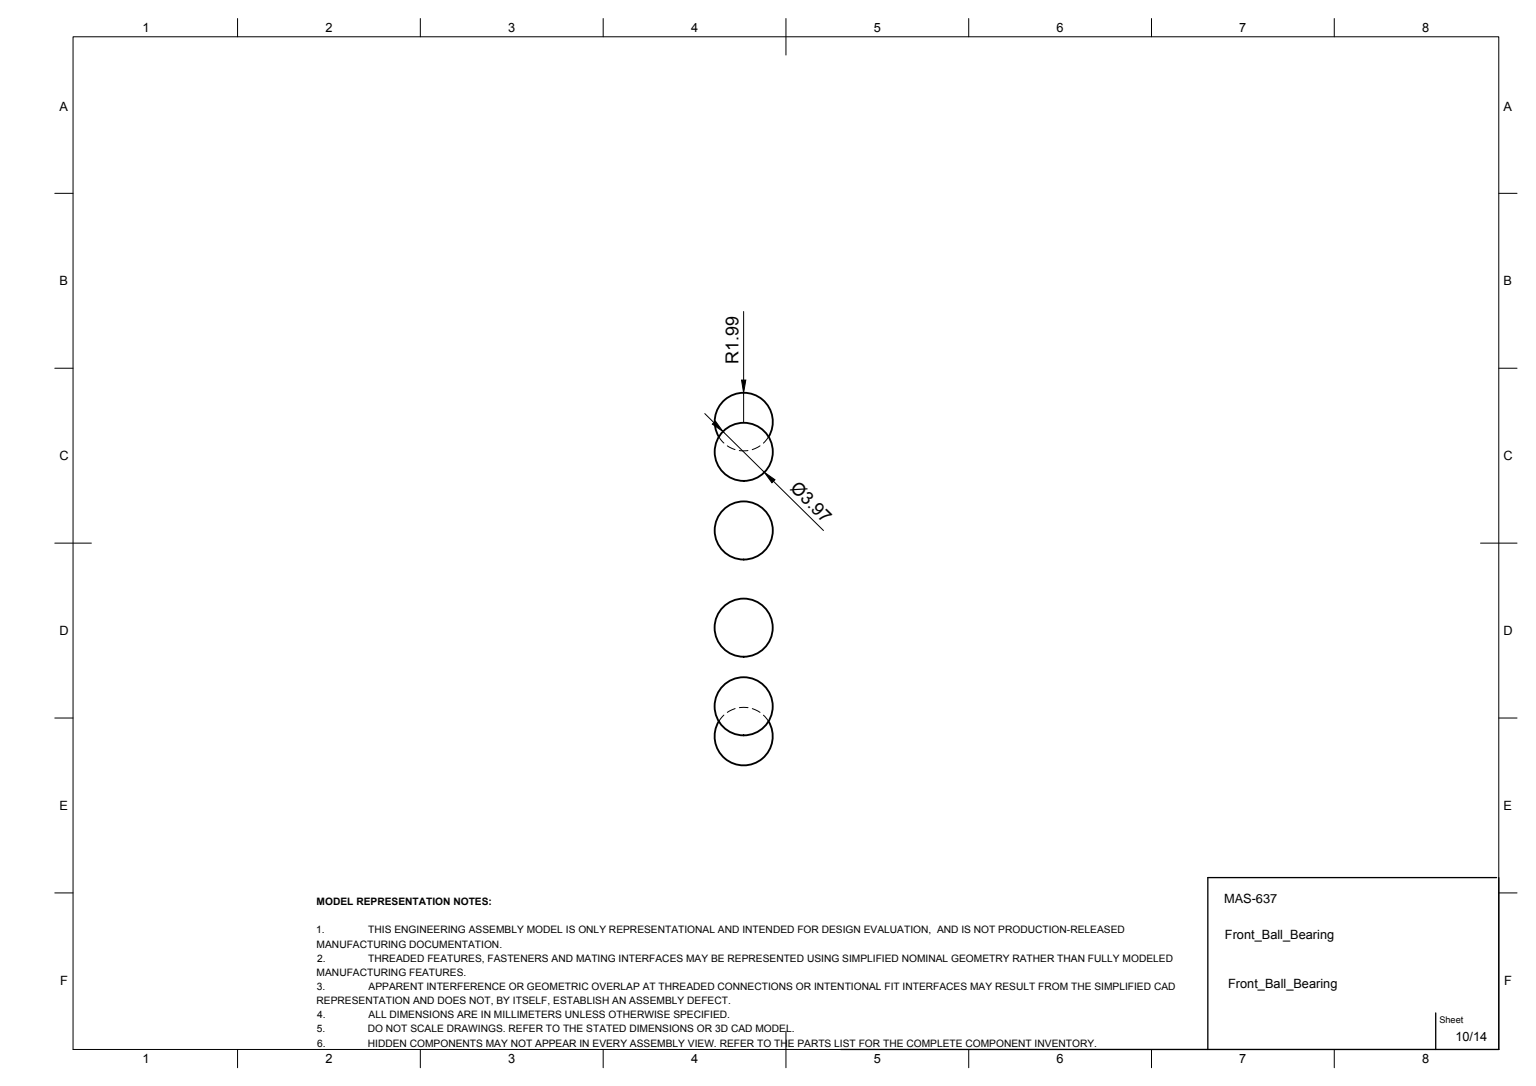
ISO-10303-21;
HEADER;
FILE_DESCRIPTION((''),'2;1');
FILE_NAME('Front_Ball_Bearing.step','2026-10-09T10:11:57-07:00',(''),(''),'','','');
FILE_SCHEMA (('AUTOMOTIVE_DESIGN { 1 0 10303 214 3 1 1 }'));
ENDSEC;
DATA;
#10=MECHANICAL_DESIGN_GEOMETRIC_PRESENTATION_REPRESENTATION('',(#133,#134,#135,#136,#137,#138,#139,#140,#141,#142),#13510);
#74=SPHERICAL_SURFACE('',#8349,1.985) ;
#75=SPHERICAL_SURFACE('',#8351,1.985) ;
#76=SPHERICAL_SURFACE('',#8353,1.985) ;
#77=SPHERICAL_SURFACE('',#8355,1.985) ;
#78=SPHERICAL_SURFACE('',#8357,1.985) ;
#79=SPHERICAL_SURFACE('',#8359,1.985) ;
#80=SPHERICAL_SURFACE('',#8361,1.985) ;
#81=SPHERICAL_SURFACE('',#8363,1.985) ;
#82=SPHERICAL_SURFACE('',#8365,1.985) ;
#83=SPHERICAL_SURFACE('',#8367,1.985) ;
#103=SHAPE_REPRESENTATION_RELATIONSHIP('SRR','None',#13573,#118) ;
#118=ADVANCED_BREP_SHAPE_REPRESENTATION('',(#165,#166,#167,#168,#169,#170,
#171,#172,#173,#174),#13505) ;
#133=STYLED_ITEM('',(#13650),#165) ;
#134=STYLED_ITEM('',(#13650),#166) ;
#135=STYLED_ITEM('',(#13650),#167) ;
#136=STYLED_ITEM('',(#13650),#168) ;
#137=STYLED_ITEM('',(#13650),#169) ;
#138=STYLED_ITEM('',(#13650),#170) ;
#139=STYLED_ITEM('',(#13650),#171) ;
#140=STYLED_ITEM('',(#13650),#172) ;
#141=STYLED_ITEM('',(#13650),#173) ;
#142=STYLED_ITEM('',(#13650),#174) ;
#165=MANIFOLD_SOLID_BREP('Body1',#7382) ;
#166=MANIFOLD_SOLID_BREP('Body2',#7383) ;
#167=MANIFOLD_SOLID_BREP('Body3',#7384) ;
#168=MANIFOLD_SOLID_BREP('Body4',#7385) ;
#169=MANIFOLD_SOLID_BREP('Body5',#7386) ;
#170=MANIFOLD_SOLID_BREP('Body6',#7387) ;
#171=MANIFOLD_SOLID_BREP('Body7',#7388) ;
#172=MANIFOLD_SOLID_BREP('Body8',#7389) ;
#173=MANIFOLD_SOLID_BREP('Body9',#7390) ;
#174=MANIFOLD_SOLID_BREP('Body10',#7391) ;
#1035=FACE_OUTER_BOUND('',#1550,.T.) ;
#1036=FACE_OUTER_BOUND('',#1551,.T.) ;
#1037=FACE_OUTER_BOUND('',#1552,.T.) ;
#1038=FACE_OUTER_BOUND('',#1553,.T.) ;
#1039=FACE_OUTER_BOUND('',#1554,.T.) ;
#1040=FACE_OUTER_BOUND('',#1555,.T.) ;
#1041=FACE_OUTER_BOUND('',#1556,.T.) ;
#1042=FACE_OUTER_BOUND('',#1557,.T.) ;
#1043=FACE_OUTER_BOUND('',#1558,.T.) ;
#1044=FACE_OUTER_BOUND('',#1559,.T.) ;
#1550=EDGE_LOOP('',(#6584,#6585)) ;
#1551=EDGE_LOOP('',(#6586,#6587)) ;
#1552=EDGE_LOOP('',(#6588,#6589)) ;
#1553=EDGE_LOOP('',(#6590,#6591)) ;
#1554=EDGE_LOOP('',(#6592,#6593)) ;
#1555=EDGE_LOOP('',(#6594,#6595)) ;
#1556=EDGE_LOOP('',(#6596,#6597)) ;
#1557=EDGE_LOOP('',(#6598,#6599)) ;
#1558=EDGE_LOOP('',(#6600,#6601)) ;
#1559=EDGE_LOOP('',(#6602,#6603)) ;
#3031=CIRCLE('',#8350,1.985) ;
#3032=CIRCLE('',#8352,1.985) ;
#3033=CIRCLE('',#8354,1.985) ;
#3034=CIRCLE('',#8356,1.985) ;
#3035=CIRCLE('',#8358,1.985) ;
#3036=CIRCLE('',#8360,1.985) ;
#3037=CIRCLE('',#8362,1.985) ;
#3038=CIRCLE('',#8364,1.985) ;
#3039=CIRCLE('',#8366,1.985) ;
#3040=CIRCLE('',#8368,1.985) ;
#3692=VERTEX_POINT('',#13123) ;
#3693=VERTEX_POINT('',#13124) ;
#3694=VERTEX_POINT('',#13127) ;
#3695=VERTEX_POINT('',#13128) ;
#3696=VERTEX_POINT('',#13131) ;
#3697=VERTEX_POINT('',#13132) ;
#3698=VERTEX_POINT('',#13135) ;
#3699=VERTEX_POINT('',#13136) ;
#3700=VERTEX_POINT('',#13139) ;
#3701=VERTEX_POINT('',#13140) ;
#3702=VERTEX_POINT('',#13143) ;
#3703=VERTEX_POINT('',#13144) ;
#3704=VERTEX_POINT('',#13147) ;
#3705=VERTEX_POINT('',#13148) ;
#3706=VERTEX_POINT('',#13151) ;
#3707=VERTEX_POINT('',#13152) ;
#3708=VERTEX_POINT('',#13155) ;
#3709=VERTEX_POINT('',#13156) ;
#3710=VERTEX_POINT('',#13159) ;
#3711=VERTEX_POINT('',#13160) ;
#4679=EDGE_CURVE('',#3692,#3693,#3031,.T.) ;
#4680=EDGE_CURVE('',#3694,#3695,#3032,.T.) ;
#4681=EDGE_CURVE('',#3696,#3697,#3033,.T.) ;
#4682=EDGE_CURVE('',#3698,#3699,#3034,.T.) ;
#4683=EDGE_CURVE('',#3700,#3701,#3035,.T.) ;
#4684=EDGE_CURVE('',#3702,#3703,#3036,.T.) ;
#4685=EDGE_CURVE('',#3704,#3705,#3037,.T.) ;
#4686=EDGE_CURVE('',#3706,#3707,#3038,.T.) ;
#4687=EDGE_CURVE('',#3708,#3709,#3039,.T.) ;
#4688=EDGE_CURVE('',#3710,#3711,#3040,.T.) ;
#6584=ORIENTED_EDGE('',*,*,#4679,.T.) ;
#6585=ORIENTED_EDGE('',*,*,#4679,.F.) ;
#6586=ORIENTED_EDGE('',*,*,#4680,.T.) ;
#6587=ORIENTED_EDGE('',*,*,#4680,.F.) ;
#6588=ORIENTED_EDGE('',*,*,#4681,.T.) ;
#6589=ORIENTED_EDGE('',*,*,#4681,.F.) ;
#6590=ORIENTED_EDGE('',*,*,#4682,.T.) ;
#6591=ORIENTED_EDGE('',*,*,#4682,.F.) ;
#6592=ORIENTED_EDGE('',*,*,#4683,.T.) ;
#6593=ORIENTED_EDGE('',*,*,#4683,.F.) ;
#6594=ORIENTED_EDGE('',*,*,#4684,.T.) ;
#6595=ORIENTED_EDGE('',*,*,#4684,.F.) ;
#6596=ORIENTED_EDGE('',*,*,#4685,.T.) ;
#6597=ORIENTED_EDGE('',*,*,#4685,.F.) ;
#6598=ORIENTED_EDGE('',*,*,#4686,.T.) ;
#6599=ORIENTED_EDGE('',*,*,#4686,.F.) ;
#6600=ORIENTED_EDGE('',*,*,#4687,.T.) ;
#6601=ORIENTED_EDGE('',*,*,#4687,.F.) ;
#6602=ORIENTED_EDGE('',*,*,#4688,.T.) ;
#6603=ORIENTED_EDGE('',*,*,#4688,.F.) ;
#7285=ADVANCED_FACE('',(#1035),#74,.T.) ;
#7286=ADVANCED_FACE('',(#1036),#75,.T.) ;
#7287=ADVANCED_FACE('',(#1037),#76,.T.) ;
#7288=ADVANCED_FACE('',(#1038),#77,.T.) ;
#7289=ADVANCED_FACE('',(#1039),#78,.T.) ;
#7290=ADVANCED_FACE('',(#1040),#79,.T.) ;
#7291=ADVANCED_FACE('',(#1041),#80,.T.) ;
#7292=ADVANCED_FACE('',(#1042),#81,.T.) ;
#7293=ADVANCED_FACE('',(#1043),#82,.T.) ;
#7294=ADVANCED_FACE('',(#1044),#83,.T.) ;
#7382=CLOSED_SHELL('',(#7285)) ;
#7383=CLOSED_SHELL('',(#7286)) ;
#7384=CLOSED_SHELL('',(#7287)) ;
#7385=CLOSED_SHELL('',(#7288)) ;
#7386=CLOSED_SHELL('',(#7289)) ;
#7387=CLOSED_SHELL('',(#7290)) ;
#7388=CLOSED_SHELL('',(#7291)) ;
#7389=CLOSED_SHELL('',(#7292)) ;
#7390=CLOSED_SHELL('',(#7293)) ;
#7391=CLOSED_SHELL('',(#7294)) ;
#8348=AXIS2_PLACEMENT_3D('',#13121,#10586,#10587) ;
#8349=AXIS2_PLACEMENT_3D('',#13122,#10588,#10589) ;
#8350=AXIS2_PLACEMENT_3D('',#13125,#10590,#10591) ;
#8351=AXIS2_PLACEMENT_3D('',#13126,#10592,#10593) ;
#8352=AXIS2_PLACEMENT_3D('',#13129,#10594,#10595) ;
#8353=AXIS2_PLACEMENT_3D('',#13130,#10596,#10597) ;
#8354=AXIS2_PLACEMENT_3D('',#13133,#10598,#10599) ;
#8355=AXIS2_PLACEMENT_3D('',#13134,#10600,#10601) ;
#8356=AXIS2_PLACEMENT_3D('',#13137,#10602,#10603) ;
#8357=AXIS2_PLACEMENT_3D('',#13138,#10604,#10605) ;
#8358=AXIS2_PLACEMENT_3D('',#13141,#10606,#10607) ;
#8359=AXIS2_PLACEMENT_3D('',#13142,#10608,#10609) ;
#8360=AXIS2_PLACEMENT_3D('',#13145,#10610,#10611) ;
#8361=AXIS2_PLACEMENT_3D('',#13146,#10612,#10613) ;
#8362=AXIS2_PLACEMENT_3D('',#13149,#10614,#10615) ;
#8363=AXIS2_PLACEMENT_3D('',#13150,#10616,#10617) ;
#8364=AXIS2_PLACEMENT_3D('',#13153,#10618,#10619) ;
#8365=AXIS2_PLACEMENT_3D('',#13154,#10620,#10621) ;
#8366=AXIS2_PLACEMENT_3D('',#13157,#10622,#10623) ;
#8367=AXIS2_PLACEMENT_3D('',#13158,#10624,#10625) ;
#8368=AXIS2_PLACEMENT_3D('',#13161,#10626,#10627) ;
#10586=DIRECTION('axis',(0.,0.,1.)) ;
#10587=DIRECTION('refdir',(1.,0.,0.)) ;
#10588=DIRECTION('center_axis',(-1.,8.80690426921701E-17,0.)) ;
#10589=DIRECTION('ref_axis',(0.,0.479425538604204,0.877582561890372)) ;
#10590=DIRECTION('center_axis',(-5.15252374060181E-17,-0.877582561890372,
0.479425538604204)) ;
#10591=DIRECTION('ref_axis',(0.,-0.479425538604204,-0.877582561890372)) ;
#10592=DIRECTION('center_axis',(-0.809016994375191,0.587785252292138,0.)) ;
#10593=DIRECTION('ref_axis',(0.281799261163818,0.387863408268351,0.877582561890324)) ;
#10594=DIRECTION('center_axis',(-0.515830087547885,-0.70997920653659,0.479425538604292)) ;
#10595=DIRECTION('ref_axis',(-0.281799261163818,-0.387863408268351,-0.877582561890324)) ;
#10596=DIRECTION('center_axis',(-0.30901699437504,0.951056516295123,0.)) ;
#10597=DIRECTION('ref_axis',(0.455960782568073,0.148150638966185,0.877582561890231)) ;
#10598=DIRECTION('center_axis',(-0.834630614072673,-0.271187925591267,0.479425538604462)) ;
#10599=DIRECTION('ref_axis',(-0.455960782568073,-0.148150638966186,-0.877582561890231)) ;
#10600=DIRECTION('center_axis',(0.30901699437504,0.951056516295123,0.)) ;
#10601=DIRECTION('ref_axis',(0.455960782568073,-0.148150638966185,0.877582561890231)) ;
#10602=DIRECTION('center_axis',(-0.834630614072673,0.271187925591267,0.479425538604462)) ;
#10603=DIRECTION('ref_axis',(-0.455960782568073,0.148150638966185,-0.877582561890231)) ;
#10604=DIRECTION('center_axis',(0.809016994375191,0.587785252292138,0.)) ;
#10605=DIRECTION('ref_axis',(0.281799261163818,-0.387863408268351,0.877582561890324)) ;
#10606=DIRECTION('center_axis',(-0.515830087547885,0.70997920653659,0.479425538604292)) ;
#10607=DIRECTION('ref_axis',(-0.281799261163818,0.387863408268351,-0.877582561890324)) ;
#10608=DIRECTION('center_axis',(1.,3.439563722283E-17,0.)) ;
#10609=DIRECTION('ref_axis',(0.,-0.479425538604204,0.877582561890372)) ;
#10610=DIRECTION('center_axis',(-5.59476301348721E-17,0.877582561890372,
0.479425538604204)) ;
#10611=DIRECTION('ref_axis',(0.,0.479425538604204,-0.877582561890372)) ;
#10612=DIRECTION('center_axis',(0.809016994375191,-0.587785252292138,0.)) ;
#10613=DIRECTION('ref_axis',(-0.281799261163818,-0.387863408268351,0.877582561890324)) ;
#10614=DIRECTION('center_axis',(0.515830087547885,0.70997920653659,0.479425538604292)) ;
#10615=DIRECTION('ref_axis',(0.281799261163818,0.387863408268351,-0.877582561890324)) ;
#10616=DIRECTION('center_axis',(0.30901699437504,-0.951056516295123,0.)) ;
#10617=DIRECTION('ref_axis',(-0.455960782568073,-0.148150638966185,0.877582561890231)) ;
#10618=DIRECTION('center_axis',(0.834630614072673,0.271187925591267,0.479425538604462)) ;
#10619=DIRECTION('ref_axis',(0.455960782568073,0.148150638966186,-0.877582561890231)) ;
#10620=DIRECTION('center_axis',(-0.30901699437504,-0.951056516295123,0.)) ;
#10621=DIRECTION('ref_axis',(-0.455960782568073,0.148150638966185,0.877582561890231)) ;
#10622=DIRECTION('center_axis',(0.834630614072673,-0.271187925591267,0.479425538604462)) ;
#10623=DIRECTION('ref_axis',(0.455960782568073,-0.148150638966185,-0.877582561890231)) ;
#10624=DIRECTION('center_axis',(-0.809016994375191,-0.587785252292138,0.)) ;
#10625=DIRECTION('ref_axis',(-0.281799261163818,0.387863408268351,0.877582561890324)) ;
#10626=DIRECTION('center_axis',(0.515830087547885,-0.70997920653659,0.479425538604292)) ;
#10627=DIRECTION('ref_axis',(0.281799261163818,-0.387863408268351,-0.877582561890324)) ;
#13121=CARTESIAN_POINT('',(0.,0.,0.)) ;
#13122=CARTESIAN_POINT('Origin',(10.75,0.,6.5)) ;
#13123=CARTESIAN_POINT('',(8.765,3.14846850272417E-17,6.5)) ;
#13124=CARTESIAN_POINT('',(12.735,-1.48029384856547E-16,6.5)) ;
#13125=CARTESIAN_POINT('Origin',(10.75,0.,6.5)) ;
#13126=CARTESIAN_POINT('Origin',(8.69693268953,-6.31869146214,6.5)) ;
#13127=CARTESIAN_POINT('',(7.09103395569525,-5.15193773634011,6.5)) ;
#13128=CARTESIAN_POINT('',(10.3028314233648,-7.48544518793989,6.5)) ;
#13129=CARTESIAN_POINT('Origin',(8.69693268953,-6.31869146214,6.5)) ;
#13130=CARTESIAN_POINT('Origin',(3.32193268953,-10.2238575502,6.5)) ;
#13131=CARTESIAN_POINT('',(2.70853395569555,-8.33601036535418,6.5)) ;
#13132=CARTESIAN_POINT('',(3.93533142336446,-12.1117047350458,6.5)) ;
#13133=CARTESIAN_POINT('Origin',(3.32193268953,-10.2238575502,6.5)) ;
#13134=CARTESIAN_POINT('Origin',(-3.32193268953,-10.2238575502,6.5)) ;
#13135=CARTESIAN_POINT('',(-2.70853395569555,-8.33601036535418,6.5)) ;
#13136=CARTESIAN_POINT('',(-3.93533142336445,-12.1117047350458,6.5)) ;
#13137=CARTESIAN_POINT('Origin',(-3.32193268953,-10.2238575502,6.5)) ;
#13138=CARTESIAN_POINT('Origin',(-8.69693268953,-6.31869146214,6.5)) ;
#13139=CARTESIAN_POINT('',(-7.09103395569525,-5.15193773634011,6.5)) ;
#13140=CARTESIAN_POINT('',(-10.3028314233648,-7.48544518793989,6.5)) ;
#13141=CARTESIAN_POINT('Origin',(-8.69693268953,-6.31869146214,6.5)) ;
#13142=CARTESIAN_POINT('Origin',(-10.75,-1.31649530908E-15,6.5)) ;
#13143=CARTESIAN_POINT('',(-8.765,-1.16076210996322E-15,6.5)) ;
#13144=CARTESIAN_POINT('',(-12.735,-1.35568380836748E-15,6.5)) ;
#13145=CARTESIAN_POINT('Origin',(-10.75,-1.31649530908E-15,6.5)) ;
#13146=CARTESIAN_POINT('Origin',(-8.69693268953,6.31869146214,6.5)) ;
#13147=CARTESIAN_POINT('',(-7.09103395569525,5.15193773634011,6.5)) ;
#13148=CARTESIAN_POINT('',(-10.3028314233648,7.48544518793989,6.5)) ;
#13149=CARTESIAN_POINT('Origin',(-8.69693268953,6.31869146214,6.5)) ;
#13150=CARTESIAN_POINT('Origin',(-3.32193268953,10.2238575502,6.5)) ;
#13151=CARTESIAN_POINT('',(-2.70853395569555,8.33601036535418,6.5)) ;
#13152=CARTESIAN_POINT('',(-3.93533142336446,12.1117047350458,6.5)) ;
#13153=CARTESIAN_POINT('Origin',(-3.32193268953,10.2238575502,6.5)) ;
#13154=CARTESIAN_POINT('Origin',(3.32193268953,10.2238575502,6.5)) ;
#13155=CARTESIAN_POINT('',(2.70853395569555,8.33601036535418,6.5)) ;
#13156=CARTESIAN_POINT('',(3.93533142336445,12.1117047350458,6.5)) ;
#13157=CARTESIAN_POINT('Origin',(3.32193268953,10.2238575502,6.5)) ;
#13158=CARTESIAN_POINT('Origin',(8.69693268953,6.31869146214,6.5)) ;
#13159=CARTESIAN_POINT('',(7.09103395569525,5.15193773634011,6.5)) ;
#13160=CARTESIAN_POINT('',(10.3028314233648,7.48544518793989,6.5)) ;
#13161=CARTESIAN_POINT('Origin',(8.69693268953,6.31869146214,6.5)) ;
#13488=UNCERTAINTY_MEASURE_WITH_UNIT(LENGTH_MEASURE(0.01),#13511,
'DISTANCE_ACCURACY_VALUE',
'Maximum model space distance between geometric entities at asserted c
onnectivities') ;
#13493=UNCERTAINTY_MEASURE_WITH_UNIT(LENGTH_MEASURE(0.01),#13511,
'DISTANCE_ACCURACY_VALUE',
'Maximum model space distance between geometric entities at asserted c
onnectivities') ;
#13505=(
GEOMETRIC_REPRESENTATION_CONTEXT(3)
GLOBAL_UNCERTAINTY_ASSIGNED_CONTEXT((#13488))
GLOBAL_UNIT_ASSIGNED_CONTEXT((#13511,#13513,#13514))
REPRESENTATION_CONTEXT('','3D')
) ;
#13510=(
GEOMETRIC_REPRESENTATION_CONTEXT(3)
GLOBAL_UNCERTAINTY_ASSIGNED_CONTEXT((#13493))
GLOBAL_UNIT_ASSIGNED_CONTEXT((#13511,#13513,#13514))
REPRESENTATION_CONTEXT('','3D')
) ;
#13511=(
LENGTH_UNIT()
NAMED_UNIT(*)
SI_UNIT(.MILLI.,.METRE.)
) ;
#13513=(
NAMED_UNIT(*)
PLANE_ANGLE_UNIT()
SI_UNIT($,.RADIAN.)
) ;
#13514=(
NAMED_UNIT(*)
SI_UNIT($,.STERADIAN.)
SOLID_ANGLE_UNIT()
) ;
#13526=SHAPE_DEFINITION_REPRESENTATION(#13542,#13573) ;
#13542=PRODUCT_DEFINITION_SHAPE('',$,#13590) ;
#13573=SHAPE_REPRESENTATION('',(#8348),#13505) ;
#13578=PRODUCT_DEFINITION_CONTEXT('part definition',#13628,'design') ;
#13590=PRODUCT_DEFINITION('Front_Ball_Bearing','Front_Ball_Bearing',#13606,
#13578) ;
#13606=PRODUCT_DEFINITION_FORMATION('',$,#13641) ;
#13628=APPLICATION_CONTEXT(
'Core Data for Automotive Mechanical Design Process') ;
#13629=PRODUCT_CONTEXT('part definition',#13628,'mechanical') ;
#13641=PRODUCT('Front_Ball_Bearing','Front_Ball_Bearing',$,(#13629)) ;
#13650=PRESENTATION_STYLE_ASSIGNMENT((#13655)) ;
#13655=SURFACE_STYLE_USAGE(.BOTH.,#13660) ;
#13660=SURFACE_SIDE_STYLE('',(#13665)) ;
#13665=SURFACE_STYLE_FILL_AREA(#13670) ;
#13670=FILL_AREA_STYLE('Opaque(144,144,144)',(#13675)) ;
#13675=FILL_AREA_STYLE_COLOUR('Opaque(144,144,144)',#13680) ;
#13680=COLOUR_RGB('Opaque(144,144,144)', 0.40784314, 0.44705882, 0.49803922) ;
ENDSEC;
END-ISO-10303-21;
